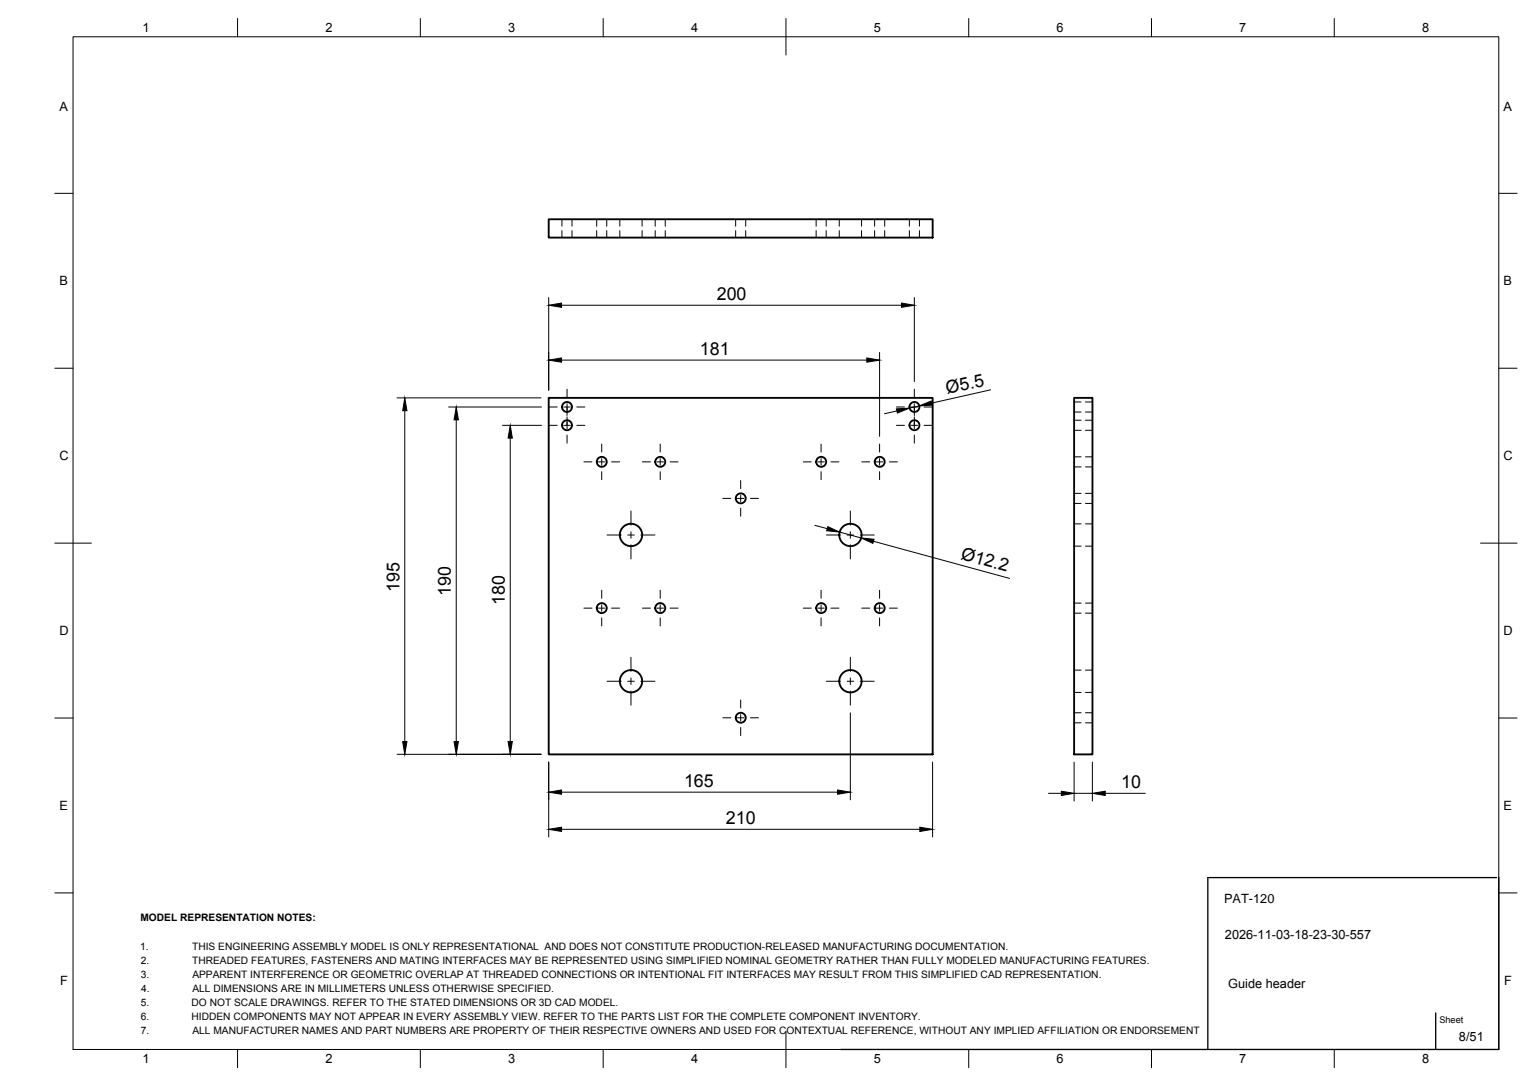
ISO-10303-21;
HEADER;
/* Generated by software containing ST-Developer
 * from STEP Tools, Inc. (www.steptools.com) 
 */

FILE_DESCRIPTION(
/* description */ ('Vibration shaker table dummy'),
/* implementation_level */ '2;1');

FILE_NAME(
/* name */ 'Guide header.step',
/* time_stamp */ '2026-10-27T10:55:14-07:00',
/* author */ (''),
/* organization */ (''),
/* preprocessor_version */ 'ST-DEVELOPER v20.2',
/* originating_system */ 'Autodesk Translation Framework v15.17.0.0',
/* authorisation */ '');

FILE_SCHEMA (('AUTOMOTIVE_DESIGN { 1 0 10303 214 3 1 1 }'));
ENDSEC;

DATA;
#10=MECHANICAL_DESIGN_GEOMETRIC_PRESENTATION_REPRESENTATION('',(#689),#22394);
#597=SHAPE_REPRESENTATION_RELATIONSHIP('SRR','None',#22643,#643);
#643=ADVANCED_BREP_SHAPE_REPRESENTATION('',(#735),#22349);
#689=STYLED_ITEM('',(#22947),#735);
#735=MANIFOLD_SOLID_BREP('Body1',#9207);
#819=FACE_BOUND('',#1946,.T.);
#820=FACE_BOUND('',#1947,.T.);
#821=FACE_BOUND('',#1948,.T.);
#822=FACE_BOUND('',#1949,.T.);
#823=FACE_BOUND('',#1950,.T.);
#824=FACE_BOUND('',#1951,.T.);
#825=FACE_BOUND('',#1952,.T.);
#826=FACE_BOUND('',#1953,.T.);
#827=FACE_BOUND('',#1954,.T.);
#828=FACE_BOUND('',#1955,.T.);
#829=FACE_BOUND('',#1956,.T.);
#830=FACE_BOUND('',#1957,.T.);
#831=FACE_BOUND('',#1958,.T.);
#832=FACE_BOUND('',#1959,.T.);
#833=FACE_BOUND('',#1960,.T.);
#834=FACE_BOUND('',#1961,.T.);
#835=FACE_BOUND('',#1962,.T.);
#836=FACE_BOUND('',#1963,.T.);
#837=FACE_BOUND('',#1965,.T.);
#838=FACE_BOUND('',#1966,.T.);
#839=FACE_BOUND('',#1967,.T.);
#840=FACE_BOUND('',#1968,.T.);
#841=FACE_BOUND('',#1969,.T.);
#842=FACE_BOUND('',#1970,.T.);
#843=FACE_BOUND('',#1971,.T.);
#844=FACE_BOUND('',#1972,.T.);
#845=FACE_BOUND('',#1973,.T.);
#846=FACE_BOUND('',#1974,.T.);
#847=FACE_BOUND('',#1975,.T.);
#848=FACE_BOUND('',#1976,.T.);
#849=FACE_BOUND('',#1977,.T.);
#850=FACE_BOUND('',#1978,.T.);
#851=FACE_BOUND('',#1979,.T.);
#852=FACE_BOUND('',#1980,.T.);
#853=FACE_BOUND('',#1981,.T.);
#854=FACE_BOUND('',#1982,.T.);
#1078=PLANE('',#9904);
#1079=PLANE('',#9905);
#1080=PLANE('',#9906);
#1081=PLANE('',#9907);
#1082=PLANE('',#9908);
#1083=PLANE('',#9909);
#1381=FACE_OUTER_BOUND('',#1923,.T.);
#1382=FACE_OUTER_BOUND('',#1924,.T.);
#1383=FACE_OUTER_BOUND('',#1925,.T.);
#1384=FACE_OUTER_BOUND('',#1926,.T.);
#1385=FACE_OUTER_BOUND('',#1927,.T.);
#1386=FACE_OUTER_BOUND('',#1928,.T.);
#1387=FACE_OUTER_BOUND('',#1929,.T.);
#1388=FACE_OUTER_BOUND('',#1930,.T.);
#1389=FACE_OUTER_BOUND('',#1931,.T.);
#1390=FACE_OUTER_BOUND('',#1932,.T.);
#1391=FACE_OUTER_BOUND('',#1933,.T.);
#1392=FACE_OUTER_BOUND('',#1934,.T.);
#1393=FACE_OUTER_BOUND('',#1935,.T.);
#1394=FACE_OUTER_BOUND('',#1936,.T.);
#1395=FACE_OUTER_BOUND('',#1937,.T.);
#1396=FACE_OUTER_BOUND('',#1938,.T.);
#1397=FACE_OUTER_BOUND('',#1939,.T.);
#1398=FACE_OUTER_BOUND('',#1940,.T.);
#1399=FACE_OUTER_BOUND('',#1941,.T.);
#1400=FACE_OUTER_BOUND('',#1942,.T.);
#1401=FACE_OUTER_BOUND('',#1943,.T.);
#1402=FACE_OUTER_BOUND('',#1944,.T.);
#1403=FACE_OUTER_BOUND('',#1945,.T.);
#1404=FACE_OUTER_BOUND('',#1964,.T.);
#1923=EDGE_LOOP('',(#6450,#6451,#6452,#6453));
#1924=EDGE_LOOP('',(#6454,#6455,#6456,#6457));
#1925=EDGE_LOOP('',(#6458,#6459,#6460,#6461));
#1926=EDGE_LOOP('',(#6462,#6463,#6464,#6465));
#1927=EDGE_LOOP('',(#6466,#6467,#6468,#6469));
#1928=EDGE_LOOP('',(#6470,#6471,#6472,#6473));
#1929=EDGE_LOOP('',(#6474,#6475,#6476,#6477));
#1930=EDGE_LOOP('',(#6478,#6479,#6480,#6481));
#1931=EDGE_LOOP('',(#6482,#6483,#6484,#6485));
#1932=EDGE_LOOP('',(#6486,#6487,#6488,#6489));
#1933=EDGE_LOOP('',(#6490,#6491,#6492,#6493));
#1934=EDGE_LOOP('',(#6494,#6495,#6496,#6497));
#1935=EDGE_LOOP('',(#6498,#6499,#6500,#6501));
#1936=EDGE_LOOP('',(#6502,#6503,#6504,#6505));
#1937=EDGE_LOOP('',(#6506,#6507,#6508,#6509));
#1938=EDGE_LOOP('',(#6510,#6511,#6512,#6513));
#1939=EDGE_LOOP('',(#6514,#6515,#6516,#6517));
#1940=EDGE_LOOP('',(#6518,#6519,#6520,#6521));
#1941=EDGE_LOOP('',(#6522,#6523,#6524,#6525));
#1942=EDGE_LOOP('',(#6526,#6527,#6528,#6529));
#1943=EDGE_LOOP('',(#6530,#6531,#6532,#6533));
#1944=EDGE_LOOP('',(#6534,#6535,#6536,#6537));
#1945=EDGE_LOOP('',(#6538,#6539,#6540,#6541));
#1946=EDGE_LOOP('',(#6542));
#1947=EDGE_LOOP('',(#6543));
#1948=EDGE_LOOP('',(#6544));
#1949=EDGE_LOOP('',(#6545));
#1950=EDGE_LOOP('',(#6546));
#1951=EDGE_LOOP('',(#6547));
#1952=EDGE_LOOP('',(#6548));
#1953=EDGE_LOOP('',(#6549));
#1954=EDGE_LOOP('',(#6550));
#1955=EDGE_LOOP('',(#6551));
#1956=EDGE_LOOP('',(#6552));
#1957=EDGE_LOOP('',(#6553));
#1958=EDGE_LOOP('',(#6554));
#1959=EDGE_LOOP('',(#6555));
#1960=EDGE_LOOP('',(#6556));
#1961=EDGE_LOOP('',(#6557));
#1962=EDGE_LOOP('',(#6558));
#1963=EDGE_LOOP('',(#6559));
#1964=EDGE_LOOP('',(#6560,#6561,#6562,#6563));
#1965=EDGE_LOOP('',(#6564));
#1966=EDGE_LOOP('',(#6565));
#1967=EDGE_LOOP('',(#6566));
#1968=EDGE_LOOP('',(#6567));
#1969=EDGE_LOOP('',(#6568));
#1970=EDGE_LOOP('',(#6569));
#1971=EDGE_LOOP('',(#6570));
#1972=EDGE_LOOP('',(#6571));
#1973=EDGE_LOOP('',(#6572));
#1974=EDGE_LOOP('',(#6573));
#1975=EDGE_LOOP('',(#6574));
#1976=EDGE_LOOP('',(#6575));
#1977=EDGE_LOOP('',(#6576));
#1978=EDGE_LOOP('',(#6577));
#1979=EDGE_LOOP('',(#6578));
#1980=EDGE_LOOP('',(#6579));
#1981=EDGE_LOOP('',(#6580));
#1982=EDGE_LOOP('',(#6581));
#2680=LINE('',#14169,#3299);
#2681=LINE('',#14175,#3300);
#2682=LINE('',#14181,#3301);
#2683=LINE('',#14187,#3302);
#2684=LINE('',#14193,#3303);
#2685=LINE('',#14199,#3304);
#2686=LINE('',#14205,#3305);
#2687=LINE('',#14211,#3306);
#2688=LINE('',#14217,#3307);
#2689=LINE('',#14223,#3308);
#2690=LINE('',#14229,#3309);
#2691=LINE('',#14235,#3310);
#2692=LINE('',#14241,#3311);
#2693=LINE('',#14247,#3312);
#2694=LINE('',#14253,#3313);
#2695=LINE('',#14259,#3314);
#2696=LINE('',#14265,#3315);
#2697=LINE('',#14271,#3316);
#2698=LINE('',#14276,#3317);
#2699=LINE('',#14278,#3318);
#2700=LINE('',#14280,#3319);
#2701=LINE('',#14281,#3320);
#2702=LINE('',#14284,#3321);
#2703=LINE('',#14286,#3322);
#2704=LINE('',#14287,#3323);
#2705=LINE('',#14290,#3324);
#2706=LINE('',#14292,#3325);
#2707=LINE('',#14293,#3326);
#2708=LINE('',#14295,#3327);
#2709=LINE('',#14296,#3328);
#3299=VECTOR('',#11192,0.275);
#3300=VECTOR('',#11199,0.275);
#3301=VECTOR('',#11206,0.275);
#3302=VECTOR('',#11213,0.275);
#3303=VECTOR('',#11220,0.275);
#3304=VECTOR('',#11227,0.275);
#3305=VECTOR('',#11234,0.275);
#3306=VECTOR('',#11241,0.275);
#3307=VECTOR('',#11248,0.275);
#3308=VECTOR('',#11255,0.275);
#3309=VECTOR('',#11262,0.275);
#3310=VECTOR('',#11269,0.275);
#3311=VECTOR('',#11276,0.275);
#3312=VECTOR('',#11283,0.275);
#3313=VECTOR('',#11290,0.61);
#3314=VECTOR('',#11297,0.61);
#3315=VECTOR('',#11304,0.61);
#3316=VECTOR('',#11311,0.61);
#3317=VECTOR('',#11316,1.);
#3318=VECTOR('',#11317,1.);
#3319=VECTOR('',#11318,1.);
#3320=VECTOR('',#11319,1.);
#3321=VECTOR('',#11322,1.);
#3322=VECTOR('',#11323,1.);
#3323=VECTOR('',#11324,1.);
#3324=VECTOR('',#11327,1.);
#3325=VECTOR('',#11328,1.);
#3326=VECTOR('',#11329,1.);
#3327=VECTOR('',#11332,1.);
#3328=VECTOR('',#11333,1.);
#3904=CIRCLE('',#9851,0.275);
#3905=CIRCLE('',#9852,0.275);
#3906=CIRCLE('',#9854,0.275);
#3907=CIRCLE('',#9855,0.275);
#3908=CIRCLE('',#9857,0.275);
#3909=CIRCLE('',#9858,0.275);
#3910=CIRCLE('',#9860,0.275);
#3911=CIRCLE('',#9861,0.275);
#3912=CIRCLE('',#9863,0.275);
#3913=CIRCLE('',#9864,0.275);
#3914=CIRCLE('',#9866,0.275);
#3915=CIRCLE('',#9867,0.275);
#3916=CIRCLE('',#9869,0.275);
#3917=CIRCLE('',#9870,0.275);
#3918=CIRCLE('',#9872,0.275);
#3919=CIRCLE('',#9873,0.275);
#3920=CIRCLE('',#9875,0.275);
#3921=CIRCLE('',#9876,0.275);
#3922=CIRCLE('',#9878,0.275);
#3923=CIRCLE('',#9879,0.275);
#3924=CIRCLE('',#9881,0.275);
#3925=CIRCLE('',#9882,0.275);
#3926=CIRCLE('',#9884,0.275);
#3927=CIRCLE('',#9885,0.275);
#3928=CIRCLE('',#9887,0.275);
#3929=CIRCLE('',#9888,0.275);
#3930=CIRCLE('',#9890,0.275);
#3931=CIRCLE('',#9891,0.275);
#3932=CIRCLE('',#9893,0.61);
#3933=CIRCLE('',#9894,0.61);
#3934=CIRCLE('',#9896,0.61);
#3935=CIRCLE('',#9897,0.61);
#3936=CIRCLE('',#9899,0.61);
#3937=CIRCLE('',#9900,0.61);
#3938=CIRCLE('',#9902,0.61);
#3939=CIRCLE('',#9903,0.61);
#4435=VERTEX_POINT('',#14166);
#4436=VERTEX_POINT('',#14168);
#4437=VERTEX_POINT('',#14172);
#4438=VERTEX_POINT('',#14174);
#4439=VERTEX_POINT('',#14178);
#4440=VERTEX_POINT('',#14180);
#4441=VERTEX_POINT('',#14184);
#4442=VERTEX_POINT('',#14186);
#4443=VERTEX_POINT('',#14190);
#4444=VERTEX_POINT('',#14192);
#4445=VERTEX_POINT('',#14196);
#4446=VERTEX_POINT('',#14198);
#4447=VERTEX_POINT('',#14202);
#4448=VERTEX_POINT('',#14204);
#4449=VERTEX_POINT('',#14208);
#4450=VERTEX_POINT('',#14210);
#4451=VERTEX_POINT('',#14214);
#4452=VERTEX_POINT('',#14216);
#4453=VERTEX_POINT('',#14220);
#4454=VERTEX_POINT('',#14222);
#4455=VERTEX_POINT('',#14226);
#4456=VERTEX_POINT('',#14228);
#4457=VERTEX_POINT('',#14232);
#4458=VERTEX_POINT('',#14234);
#4459=VERTEX_POINT('',#14238);
#4460=VERTEX_POINT('',#14240);
#4461=VERTEX_POINT('',#14244);
#4462=VERTEX_POINT('',#14246);
#4463=VERTEX_POINT('',#14250);
#4464=VERTEX_POINT('',#14252);
#4465=VERTEX_POINT('',#14256);
#4466=VERTEX_POINT('',#14258);
#4467=VERTEX_POINT('',#14262);
#4468=VERTEX_POINT('',#14264);
#4469=VERTEX_POINT('',#14268);
#4470=VERTEX_POINT('',#14270);
#4471=VERTEX_POINT('',#14274);
#4472=VERTEX_POINT('',#14275);
#4473=VERTEX_POINT('',#14277);
#4474=VERTEX_POINT('',#14279);
#4475=VERTEX_POINT('',#14283);
#4476=VERTEX_POINT('',#14285);
#4477=VERTEX_POINT('',#14289);
#4478=VERTEX_POINT('',#14291);
#5218=EDGE_CURVE('',#4435,#4435,#3904,.T.);
#5219=EDGE_CURVE('',#4435,#4436,#2680,.T.);
#5220=EDGE_CURVE('',#4436,#4436,#3905,.T.);
#5221=EDGE_CURVE('',#4437,#4437,#3906,.T.);
#5222=EDGE_CURVE('',#4437,#4438,#2681,.T.);
#5223=EDGE_CURVE('',#4438,#4438,#3907,.T.);
#5224=EDGE_CURVE('',#4439,#4439,#3908,.T.);
#5225=EDGE_CURVE('',#4439,#4440,#2682,.T.);
#5226=EDGE_CURVE('',#4440,#4440,#3909,.T.);
#5227=EDGE_CURVE('',#4441,#4441,#3910,.T.);
#5228=EDGE_CURVE('',#4441,#4442,#2683,.T.);
#5229=EDGE_CURVE('',#4442,#4442,#3911,.T.);
#5230=EDGE_CURVE('',#4443,#4443,#3912,.T.);
#5231=EDGE_CURVE('',#4443,#4444,#2684,.T.);
#5232=EDGE_CURVE('',#4444,#4444,#3913,.T.);
#5233=EDGE_CURVE('',#4445,#4445,#3914,.T.);
#5234=EDGE_CURVE('',#4445,#4446,#2685,.T.);
#5235=EDGE_CURVE('',#4446,#4446,#3915,.T.);
#5236=EDGE_CURVE('',#4447,#4447,#3916,.T.);
#5237=EDGE_CURVE('',#4447,#4448,#2686,.T.);
#5238=EDGE_CURVE('',#4448,#4448,#3917,.T.);
#5239=EDGE_CURVE('',#4449,#4449,#3918,.T.);
#5240=EDGE_CURVE('',#4449,#4450,#2687,.T.);
#5241=EDGE_CURVE('',#4450,#4450,#3919,.T.);
#5242=EDGE_CURVE('',#4451,#4451,#3920,.T.);
#5243=EDGE_CURVE('',#4451,#4452,#2688,.T.);
#5244=EDGE_CURVE('',#4452,#4452,#3921,.T.);
#5245=EDGE_CURVE('',#4453,#4453,#3922,.T.);
#5246=EDGE_CURVE('',#4453,#4454,#2689,.T.);
#5247=EDGE_CURVE('',#4454,#4454,#3923,.T.);
#5248=EDGE_CURVE('',#4455,#4455,#3924,.T.);
#5249=EDGE_CURVE('',#4455,#4456,#2690,.T.);
#5250=EDGE_CURVE('',#4456,#4456,#3925,.T.);
#5251=EDGE_CURVE('',#4457,#4457,#3926,.T.);
#5252=EDGE_CURVE('',#4457,#4458,#2691,.T.);
#5253=EDGE_CURVE('',#4458,#4458,#3927,.T.);
#5254=EDGE_CURVE('',#4459,#4459,#3928,.T.);
#5255=EDGE_CURVE('',#4459,#4460,#2692,.T.);
#5256=EDGE_CURVE('',#4460,#4460,#3929,.T.);
#5257=EDGE_CURVE('',#4461,#4461,#3930,.T.);
#5258=EDGE_CURVE('',#4461,#4462,#2693,.T.);
#5259=EDGE_CURVE('',#4462,#4462,#3931,.T.);
#5260=EDGE_CURVE('',#4463,#4463,#3932,.T.);
#5261=EDGE_CURVE('',#4463,#4464,#2694,.T.);
#5262=EDGE_CURVE('',#4464,#4464,#3933,.T.);
#5263=EDGE_CURVE('',#4465,#4465,#3934,.T.);
#5264=EDGE_CURVE('',#4465,#4466,#2695,.T.);
#5265=EDGE_CURVE('',#4466,#4466,#3935,.T.);
#5266=EDGE_CURVE('',#4467,#4467,#3936,.T.);
#5267=EDGE_CURVE('',#4467,#4468,#2696,.T.);
#5268=EDGE_CURVE('',#4468,#4468,#3937,.T.);
#5269=EDGE_CURVE('',#4469,#4469,#3938,.T.);
#5270=EDGE_CURVE('',#4469,#4470,#2697,.T.);
#5271=EDGE_CURVE('',#4470,#4470,#3939,.T.);
#5272=EDGE_CURVE('',#4471,#4472,#2698,.T.);
#5273=EDGE_CURVE('',#4472,#4473,#2699,.T.);
#5274=EDGE_CURVE('',#4474,#4473,#2700,.T.);
#5275=EDGE_CURVE('',#4471,#4474,#2701,.T.);
#5276=EDGE_CURVE('',#4475,#4471,#2702,.T.);
#5277=EDGE_CURVE('',#4476,#4474,#2703,.T.);
#5278=EDGE_CURVE('',#4475,#4476,#2704,.T.);
#5279=EDGE_CURVE('',#4477,#4475,#2705,.T.);
#5280=EDGE_CURVE('',#4478,#4476,#2706,.T.);
#5281=EDGE_CURVE('',#4477,#4478,#2707,.T.);
#5282=EDGE_CURVE('',#4472,#4477,#2708,.T.);
#5283=EDGE_CURVE('',#4473,#4478,#2709,.T.);
#6450=ORIENTED_EDGE('',*,*,#5218,.F.);
#6451=ORIENTED_EDGE('',*,*,#5219,.T.);
#6452=ORIENTED_EDGE('',*,*,#5220,.F.);
#6453=ORIENTED_EDGE('',*,*,#5219,.F.);
#6454=ORIENTED_EDGE('',*,*,#5221,.F.);
#6455=ORIENTED_EDGE('',*,*,#5222,.T.);
#6456=ORIENTED_EDGE('',*,*,#5223,.F.);
#6457=ORIENTED_EDGE('',*,*,#5222,.F.);
#6458=ORIENTED_EDGE('',*,*,#5224,.F.);
#6459=ORIENTED_EDGE('',*,*,#5225,.T.);
#6460=ORIENTED_EDGE('',*,*,#5226,.F.);
#6461=ORIENTED_EDGE('',*,*,#5225,.F.);
#6462=ORIENTED_EDGE('',*,*,#5227,.F.);
#6463=ORIENTED_EDGE('',*,*,#5228,.T.);
#6464=ORIENTED_EDGE('',*,*,#5229,.F.);
#6465=ORIENTED_EDGE('',*,*,#5228,.F.);
#6466=ORIENTED_EDGE('',*,*,#5230,.F.);
#6467=ORIENTED_EDGE('',*,*,#5231,.T.);
#6468=ORIENTED_EDGE('',*,*,#5232,.F.);
#6469=ORIENTED_EDGE('',*,*,#5231,.F.);
#6470=ORIENTED_EDGE('',*,*,#5233,.F.);
#6471=ORIENTED_EDGE('',*,*,#5234,.T.);
#6472=ORIENTED_EDGE('',*,*,#5235,.F.);
#6473=ORIENTED_EDGE('',*,*,#5234,.F.);
#6474=ORIENTED_EDGE('',*,*,#5236,.F.);
#6475=ORIENTED_EDGE('',*,*,#5237,.T.);
#6476=ORIENTED_EDGE('',*,*,#5238,.F.);
#6477=ORIENTED_EDGE('',*,*,#5237,.F.);
#6478=ORIENTED_EDGE('',*,*,#5239,.F.);
#6479=ORIENTED_EDGE('',*,*,#5240,.T.);
#6480=ORIENTED_EDGE('',*,*,#5241,.F.);
#6481=ORIENTED_EDGE('',*,*,#5240,.F.);
#6482=ORIENTED_EDGE('',*,*,#5242,.F.);
#6483=ORIENTED_EDGE('',*,*,#5243,.T.);
#6484=ORIENTED_EDGE('',*,*,#5244,.F.);
#6485=ORIENTED_EDGE('',*,*,#5243,.F.);
#6486=ORIENTED_EDGE('',*,*,#5245,.F.);
#6487=ORIENTED_EDGE('',*,*,#5246,.T.);
#6488=ORIENTED_EDGE('',*,*,#5247,.F.);
#6489=ORIENTED_EDGE('',*,*,#5246,.F.);
#6490=ORIENTED_EDGE('',*,*,#5248,.F.);
#6491=ORIENTED_EDGE('',*,*,#5249,.T.);
#6492=ORIENTED_EDGE('',*,*,#5250,.F.);
#6493=ORIENTED_EDGE('',*,*,#5249,.F.);
#6494=ORIENTED_EDGE('',*,*,#5251,.F.);
#6495=ORIENTED_EDGE('',*,*,#5252,.T.);
#6496=ORIENTED_EDGE('',*,*,#5253,.F.);
#6497=ORIENTED_EDGE('',*,*,#5252,.F.);
#6498=ORIENTED_EDGE('',*,*,#5254,.F.);
#6499=ORIENTED_EDGE('',*,*,#5255,.T.);
#6500=ORIENTED_EDGE('',*,*,#5256,.F.);
#6501=ORIENTED_EDGE('',*,*,#5255,.F.);
#6502=ORIENTED_EDGE('',*,*,#5257,.F.);
#6503=ORIENTED_EDGE('',*,*,#5258,.T.);
#6504=ORIENTED_EDGE('',*,*,#5259,.F.);
#6505=ORIENTED_EDGE('',*,*,#5258,.F.);
#6506=ORIENTED_EDGE('',*,*,#5260,.F.);
#6507=ORIENTED_EDGE('',*,*,#5261,.T.);
#6508=ORIENTED_EDGE('',*,*,#5262,.F.);
#6509=ORIENTED_EDGE('',*,*,#5261,.F.);
#6510=ORIENTED_EDGE('',*,*,#5263,.F.);
#6511=ORIENTED_EDGE('',*,*,#5264,.T.);
#6512=ORIENTED_EDGE('',*,*,#5265,.F.);
#6513=ORIENTED_EDGE('',*,*,#5264,.F.);
#6514=ORIENTED_EDGE('',*,*,#5266,.F.);
#6515=ORIENTED_EDGE('',*,*,#5267,.T.);
#6516=ORIENTED_EDGE('',*,*,#5268,.F.);
#6517=ORIENTED_EDGE('',*,*,#5267,.F.);
#6518=ORIENTED_EDGE('',*,*,#5269,.F.);
#6519=ORIENTED_EDGE('',*,*,#5270,.T.);
#6520=ORIENTED_EDGE('',*,*,#5271,.F.);
#6521=ORIENTED_EDGE('',*,*,#5270,.F.);
#6522=ORIENTED_EDGE('',*,*,#5272,.T.);
#6523=ORIENTED_EDGE('',*,*,#5273,.T.);
#6524=ORIENTED_EDGE('',*,*,#5274,.F.);
#6525=ORIENTED_EDGE('',*,*,#5275,.F.);
#6526=ORIENTED_EDGE('',*,*,#5276,.T.);
#6527=ORIENTED_EDGE('',*,*,#5275,.T.);
#6528=ORIENTED_EDGE('',*,*,#5277,.F.);
#6529=ORIENTED_EDGE('',*,*,#5278,.F.);
#6530=ORIENTED_EDGE('',*,*,#5279,.T.);
#6531=ORIENTED_EDGE('',*,*,#5278,.T.);
#6532=ORIENTED_EDGE('',*,*,#5280,.F.);
#6533=ORIENTED_EDGE('',*,*,#5281,.F.);
#6534=ORIENTED_EDGE('',*,*,#5282,.T.);
#6535=ORIENTED_EDGE('',*,*,#5281,.T.);
#6536=ORIENTED_EDGE('',*,*,#5283,.F.);
#6537=ORIENTED_EDGE('',*,*,#5273,.F.);
#6538=ORIENTED_EDGE('',*,*,#5283,.T.);
#6539=ORIENTED_EDGE('',*,*,#5280,.T.);
#6540=ORIENTED_EDGE('',*,*,#5277,.T.);
#6541=ORIENTED_EDGE('',*,*,#5274,.T.);
#6542=ORIENTED_EDGE('',*,*,#5223,.T.);
#6543=ORIENTED_EDGE('',*,*,#5232,.T.);
#6544=ORIENTED_EDGE('',*,*,#5235,.T.);
#6545=ORIENTED_EDGE('',*,*,#5244,.T.);
#6546=ORIENTED_EDGE('',*,*,#5247,.T.);
#6547=ORIENTED_EDGE('',*,*,#5271,.T.);
#6548=ORIENTED_EDGE('',*,*,#5268,.T.);
#6549=ORIENTED_EDGE('',*,*,#5265,.T.);
#6550=ORIENTED_EDGE('',*,*,#5262,.T.);
#6551=ORIENTED_EDGE('',*,*,#5259,.T.);
#6552=ORIENTED_EDGE('',*,*,#5256,.T.);
#6553=ORIENTED_EDGE('',*,*,#5253,.T.);
#6554=ORIENTED_EDGE('',*,*,#5250,.T.);
#6555=ORIENTED_EDGE('',*,*,#5241,.T.);
#6556=ORIENTED_EDGE('',*,*,#5238,.T.);
#6557=ORIENTED_EDGE('',*,*,#5229,.T.);
#6558=ORIENTED_EDGE('',*,*,#5226,.T.);
#6559=ORIENTED_EDGE('',*,*,#5220,.T.);
#6560=ORIENTED_EDGE('',*,*,#5282,.F.);
#6561=ORIENTED_EDGE('',*,*,#5272,.F.);
#6562=ORIENTED_EDGE('',*,*,#5276,.F.);
#6563=ORIENTED_EDGE('',*,*,#5279,.F.);
#6564=ORIENTED_EDGE('',*,*,#5221,.T.);
#6565=ORIENTED_EDGE('',*,*,#5230,.T.);
#6566=ORIENTED_EDGE('',*,*,#5233,.T.);
#6567=ORIENTED_EDGE('',*,*,#5242,.T.);
#6568=ORIENTED_EDGE('',*,*,#5245,.T.);
#6569=ORIENTED_EDGE('',*,*,#5269,.T.);
#6570=ORIENTED_EDGE('',*,*,#5266,.T.);
#6571=ORIENTED_EDGE('',*,*,#5263,.T.);
#6572=ORIENTED_EDGE('',*,*,#5260,.T.);
#6573=ORIENTED_EDGE('',*,*,#5257,.T.);
#6574=ORIENTED_EDGE('',*,*,#5254,.T.);
#6575=ORIENTED_EDGE('',*,*,#5251,.T.);
#6576=ORIENTED_EDGE('',*,*,#5248,.T.);
#6577=ORIENTED_EDGE('',*,*,#5239,.T.);
#6578=ORIENTED_EDGE('',*,*,#5236,.T.);
#6579=ORIENTED_EDGE('',*,*,#5227,.T.);
#6580=ORIENTED_EDGE('',*,*,#5224,.T.);
#6581=ORIENTED_EDGE('',*,*,#5218,.T.);
#8528=CYLINDRICAL_SURFACE('',#9850,0.275);
#8529=CYLINDRICAL_SURFACE('',#9853,0.275);
#8530=CYLINDRICAL_SURFACE('',#9856,0.275);
#8531=CYLINDRICAL_SURFACE('',#9859,0.275);
#8532=CYLINDRICAL_SURFACE('',#9862,0.275);
#8533=CYLINDRICAL_SURFACE('',#9865,0.275);
#8534=CYLINDRICAL_SURFACE('',#9868,0.275);
#8535=CYLINDRICAL_SURFACE('',#9871,0.275);
#8536=CYLINDRICAL_SURFACE('',#9874,0.275);
#8537=CYLINDRICAL_SURFACE('',#9877,0.275);
#8538=CYLINDRICAL_SURFACE('',#9880,0.275);
#8539=CYLINDRICAL_SURFACE('',#9883,0.275);
#8540=CYLINDRICAL_SURFACE('',#9886,0.275);
#8541=CYLINDRICAL_SURFACE('',#9889,0.275);
#8542=CYLINDRICAL_SURFACE('',#9892,0.61);
#8543=CYLINDRICAL_SURFACE('',#9895,0.61);
#8544=CYLINDRICAL_SURFACE('',#9898,0.61);
#8545=CYLINDRICAL_SURFACE('',#9901,0.61);
#8746=ADVANCED_FACE('',(#1381),#8528,.F.);
#8747=ADVANCED_FACE('',(#1382),#8529,.F.);
#8748=ADVANCED_FACE('',(#1383),#8530,.F.);
#8749=ADVANCED_FACE('',(#1384),#8531,.F.);
#8750=ADVANCED_FACE('',(#1385),#8532,.F.);
#8751=ADVANCED_FACE('',(#1386),#8533,.F.);
#8752=ADVANCED_FACE('',(#1387),#8534,.F.);
#8753=ADVANCED_FACE('',(#1388),#8535,.F.);
#8754=ADVANCED_FACE('',(#1389),#8536,.F.);
#8755=ADVANCED_FACE('',(#1390),#8537,.F.);
#8756=ADVANCED_FACE('',(#1391),#8538,.F.);
#8757=ADVANCED_FACE('',(#1392),#8539,.F.);
#8758=ADVANCED_FACE('',(#1393),#8540,.F.);
#8759=ADVANCED_FACE('',(#1394),#8541,.F.);
#8760=ADVANCED_FACE('',(#1395),#8542,.F.);
#8761=ADVANCED_FACE('',(#1396),#8543,.F.);
#8762=ADVANCED_FACE('',(#1397),#8544,.F.);
#8763=ADVANCED_FACE('',(#1398),#8545,.F.);
#8764=ADVANCED_FACE('',(#1399),#1078,.T.);
#8765=ADVANCED_FACE('',(#1400),#1079,.T.);
#8766=ADVANCED_FACE('',(#1401),#1080,.T.);
#8767=ADVANCED_FACE('',(#1402),#1081,.T.);
#8768=ADVANCED_FACE('',(#1403,#819,#820,#821,#822,#823,#824,#825,#826,#827,
#828,#829,#830,#831,#832,#833,#834,#835,#836),#1082,.T.);
#8769=ADVANCED_FACE('',(#1404,#837,#838,#839,#840,#841,#842,#843,#844,#845,
#846,#847,#848,#849,#850,#851,#852,#853,#854),#1083,.F.);
#9207=CLOSED_SHELL('',(#8746,#8747,#8748,#8749,#8750,#8751,#8752,#8753,
#8754,#8755,#8756,#8757,#8758,#8759,#8760,#8761,#8762,#8763,#8764,#8765,
#8766,#8767,#8768,#8769));
#9849=AXIS2_PLACEMENT_3D('',#14164,#11186,#11187);
#9850=AXIS2_PLACEMENT_3D('',#14165,#11188,#11189);
#9851=AXIS2_PLACEMENT_3D('',#14167,#11190,#11191);
#9852=AXIS2_PLACEMENT_3D('',#14170,#11193,#11194);
#9853=AXIS2_PLACEMENT_3D('',#14171,#11195,#11196);
#9854=AXIS2_PLACEMENT_3D('',#14173,#11197,#11198);
#9855=AXIS2_PLACEMENT_3D('',#14176,#11200,#11201);
#9856=AXIS2_PLACEMENT_3D('',#14177,#11202,#11203);
#9857=AXIS2_PLACEMENT_3D('',#14179,#11204,#11205);
#9858=AXIS2_PLACEMENT_3D('',#14182,#11207,#11208);
#9859=AXIS2_PLACEMENT_3D('',#14183,#11209,#11210);
#9860=AXIS2_PLACEMENT_3D('',#14185,#11211,#11212);
#9861=AXIS2_PLACEMENT_3D('',#14188,#11214,#11215);
#9862=AXIS2_PLACEMENT_3D('',#14189,#11216,#11217);
#9863=AXIS2_PLACEMENT_3D('',#14191,#11218,#11219);
#9864=AXIS2_PLACEMENT_3D('',#14194,#11221,#11222);
#9865=AXIS2_PLACEMENT_3D('',#14195,#11223,#11224);
#9866=AXIS2_PLACEMENT_3D('',#14197,#11225,#11226);
#9867=AXIS2_PLACEMENT_3D('',#14200,#11228,#11229);
#9868=AXIS2_PLACEMENT_3D('',#14201,#11230,#11231);
#9869=AXIS2_PLACEMENT_3D('',#14203,#11232,#11233);
#9870=AXIS2_PLACEMENT_3D('',#14206,#11235,#11236);
#9871=AXIS2_PLACEMENT_3D('',#14207,#11237,#11238);
#9872=AXIS2_PLACEMENT_3D('',#14209,#11239,#11240);
#9873=AXIS2_PLACEMENT_3D('',#14212,#11242,#11243);
#9874=AXIS2_PLACEMENT_3D('',#14213,#11244,#11245);
#9875=AXIS2_PLACEMENT_3D('',#14215,#11246,#11247);
#9876=AXIS2_PLACEMENT_3D('',#14218,#11249,#11250);
#9877=AXIS2_PLACEMENT_3D('',#14219,#11251,#11252);
#9878=AXIS2_PLACEMENT_3D('',#14221,#11253,#11254);
#9879=AXIS2_PLACEMENT_3D('',#14224,#11256,#11257);
#9880=AXIS2_PLACEMENT_3D('',#14225,#11258,#11259);
#9881=AXIS2_PLACEMENT_3D('',#14227,#11260,#11261);
#9882=AXIS2_PLACEMENT_3D('',#14230,#11263,#11264);
#9883=AXIS2_PLACEMENT_3D('',#14231,#11265,#11266);
#9884=AXIS2_PLACEMENT_3D('',#14233,#11267,#11268);
#9885=AXIS2_PLACEMENT_3D('',#14236,#11270,#11271);
#9886=AXIS2_PLACEMENT_3D('',#14237,#11272,#11273);
#9887=AXIS2_PLACEMENT_3D('',#14239,#11274,#11275);
#9888=AXIS2_PLACEMENT_3D('',#14242,#11277,#11278);
#9889=AXIS2_PLACEMENT_3D('',#14243,#11279,#11280);
#9890=AXIS2_PLACEMENT_3D('',#14245,#11281,#11282);
#9891=AXIS2_PLACEMENT_3D('',#14248,#11284,#11285);
#9892=AXIS2_PLACEMENT_3D('',#14249,#11286,#11287);
#9893=AXIS2_PLACEMENT_3D('',#14251,#11288,#11289);
#9894=AXIS2_PLACEMENT_3D('',#14254,#11291,#11292);
#9895=AXIS2_PLACEMENT_3D('',#14255,#11293,#11294);
#9896=AXIS2_PLACEMENT_3D('',#14257,#11295,#11296);
#9897=AXIS2_PLACEMENT_3D('',#14260,#11298,#11299);
#9898=AXIS2_PLACEMENT_3D('',#14261,#11300,#11301);
#9899=AXIS2_PLACEMENT_3D('',#14263,#11302,#11303);
#9900=AXIS2_PLACEMENT_3D('',#14266,#11305,#11306);
#9901=AXIS2_PLACEMENT_3D('',#14267,#11307,#11308);
#9902=AXIS2_PLACEMENT_3D('',#14269,#11309,#11310);
#9903=AXIS2_PLACEMENT_3D('',#14272,#11312,#11313);
#9904=AXIS2_PLACEMENT_3D('',#14273,#11314,#11315);
#9905=AXIS2_PLACEMENT_3D('',#14282,#11320,#11321);
#9906=AXIS2_PLACEMENT_3D('',#14288,#11325,#11326);
#9907=AXIS2_PLACEMENT_3D('',#14294,#11330,#11331);
#9908=AXIS2_PLACEMENT_3D('',#14297,#11334,#11335);
#9909=AXIS2_PLACEMENT_3D('',#14298,#11336,#11337);
#11186=DIRECTION('axis',(0.,0.,1.));
#11187=DIRECTION('refdir',(1.,0.,0.));
#11188=DIRECTION('center_axis',(0.,0.,1.));
#11189=DIRECTION('ref_axis',(1.,0.,0.));
#11190=DIRECTION('center_axis',(0.,0.,1.));
#11191=DIRECTION('ref_axis',(1.,0.,0.));
#11192=DIRECTION('',(0.,0.,1.));
#11193=DIRECTION('center_axis',(0.,0.,-1.));
#11194=DIRECTION('ref_axis',(1.,0.,0.));
#11195=DIRECTION('center_axis',(0.,0.,1.));
#11196=DIRECTION('ref_axis',(1.,0.,0.));
#11197=DIRECTION('center_axis',(0.,0.,1.));
#11198=DIRECTION('ref_axis',(1.,0.,0.));
#11199=DIRECTION('',(0.,0.,1.));
#11200=DIRECTION('center_axis',(0.,0.,-1.));
#11201=DIRECTION('ref_axis',(1.,0.,0.));
#11202=DIRECTION('center_axis',(0.,0.,1.));
#11203=DIRECTION('ref_axis',(1.,0.,0.));
#11204=DIRECTION('center_axis',(0.,0.,1.));
#11205=DIRECTION('ref_axis',(1.,0.,0.));
#11206=DIRECTION('',(0.,0.,1.));
#11207=DIRECTION('center_axis',(0.,0.,-1.));
#11208=DIRECTION('ref_axis',(1.,0.,0.));
#11209=DIRECTION('center_axis',(0.,0.,1.));
#11210=DIRECTION('ref_axis',(1.,0.,0.));
#11211=DIRECTION('center_axis',(0.,0.,1.));
#11212=DIRECTION('ref_axis',(1.,0.,0.));
#11213=DIRECTION('',(0.,0.,1.));
#11214=DIRECTION('center_axis',(0.,0.,-1.));
#11215=DIRECTION('ref_axis',(1.,0.,0.));
#11216=DIRECTION('center_axis',(0.,0.,1.));
#11217=DIRECTION('ref_axis',(1.,0.,0.));
#11218=DIRECTION('center_axis',(0.,0.,1.));
#11219=DIRECTION('ref_axis',(1.,0.,0.));
#11220=DIRECTION('',(0.,0.,1.));
#11221=DIRECTION('center_axis',(0.,0.,-1.));
#11222=DIRECTION('ref_axis',(1.,0.,0.));
#11223=DIRECTION('center_axis',(0.,0.,1.));
#11224=DIRECTION('ref_axis',(1.,0.,0.));
#11225=DIRECTION('center_axis',(0.,0.,1.));
#11226=DIRECTION('ref_axis',(1.,0.,0.));
#11227=DIRECTION('',(0.,0.,1.));
#11228=DIRECTION('center_axis',(0.,0.,-1.));
#11229=DIRECTION('ref_axis',(1.,0.,0.));
#11230=DIRECTION('center_axis',(0.,0.,1.));
#11231=DIRECTION('ref_axis',(1.,0.,0.));
#11232=DIRECTION('center_axis',(0.,0.,1.));
#11233=DIRECTION('ref_axis',(1.,0.,0.));
#11234=DIRECTION('',(0.,0.,1.));
#11235=DIRECTION('center_axis',(0.,0.,-1.));
#11236=DIRECTION('ref_axis',(1.,0.,0.));
#11237=DIRECTION('center_axis',(0.,0.,1.));
#11238=DIRECTION('ref_axis',(1.,0.,0.));
#11239=DIRECTION('center_axis',(0.,0.,1.));
#11240=DIRECTION('ref_axis',(1.,0.,0.));
#11241=DIRECTION('',(0.,0.,1.));
#11242=DIRECTION('center_axis',(0.,0.,-1.));
#11243=DIRECTION('ref_axis',(1.,0.,0.));
#11244=DIRECTION('center_axis',(0.,0.,1.));
#11245=DIRECTION('ref_axis',(1.,0.,0.));
#11246=DIRECTION('center_axis',(0.,0.,1.));
#11247=DIRECTION('ref_axis',(1.,0.,0.));
#11248=DIRECTION('',(0.,0.,1.));
#11249=DIRECTION('center_axis',(0.,0.,-1.));
#11250=DIRECTION('ref_axis',(1.,0.,0.));
#11251=DIRECTION('center_axis',(0.,0.,1.));
#11252=DIRECTION('ref_axis',(1.,0.,0.));
#11253=DIRECTION('center_axis',(0.,0.,1.));
#11254=DIRECTION('ref_axis',(1.,0.,0.));
#11255=DIRECTION('',(0.,0.,1.));
#11256=DIRECTION('center_axis',(0.,0.,-1.));
#11257=DIRECTION('ref_axis',(1.,0.,0.));
#11258=DIRECTION('center_axis',(0.,0.,1.));
#11259=DIRECTION('ref_axis',(1.,0.,0.));
#11260=DIRECTION('center_axis',(0.,0.,1.));
#11261=DIRECTION('ref_axis',(1.,0.,0.));
#11262=DIRECTION('',(0.,0.,1.));
#11263=DIRECTION('center_axis',(0.,0.,-1.));
#11264=DIRECTION('ref_axis',(1.,0.,0.));
#11265=DIRECTION('center_axis',(0.,0.,1.));
#11266=DIRECTION('ref_axis',(1.,0.,0.));
#11267=DIRECTION('center_axis',(0.,0.,1.));
#11268=DIRECTION('ref_axis',(1.,0.,0.));
#11269=DIRECTION('',(0.,0.,1.));
#11270=DIRECTION('center_axis',(0.,0.,-1.));
#11271=DIRECTION('ref_axis',(1.,0.,0.));
#11272=DIRECTION('center_axis',(0.,0.,1.));
#11273=DIRECTION('ref_axis',(1.,0.,0.));
#11274=DIRECTION('center_axis',(0.,0.,1.));
#11275=DIRECTION('ref_axis',(1.,0.,0.));
#11276=DIRECTION('',(0.,0.,1.));
#11277=DIRECTION('center_axis',(0.,0.,-1.));
#11278=DIRECTION('ref_axis',(1.,0.,0.));
#11279=DIRECTION('center_axis',(0.,0.,1.));
#11280=DIRECTION('ref_axis',(1.,0.,0.));
#11281=DIRECTION('center_axis',(0.,0.,1.));
#11282=DIRECTION('ref_axis',(1.,0.,0.));
#11283=DIRECTION('',(0.,0.,1.));
#11284=DIRECTION('center_axis',(0.,0.,-1.));
#11285=DIRECTION('ref_axis',(1.,0.,0.));
#11286=DIRECTION('center_axis',(0.,0.,1.));
#11287=DIRECTION('ref_axis',(1.,0.,0.));
#11288=DIRECTION('center_axis',(0.,0.,1.));
#11289=DIRECTION('ref_axis',(1.,0.,0.));
#11290=DIRECTION('',(0.,0.,1.));
#11291=DIRECTION('center_axis',(0.,0.,-1.));
#11292=DIRECTION('ref_axis',(1.,0.,0.));
#11293=DIRECTION('center_axis',(0.,0.,1.));
#11294=DIRECTION('ref_axis',(1.,0.,0.));
#11295=DIRECTION('center_axis',(0.,0.,1.));
#11296=DIRECTION('ref_axis',(1.,0.,0.));
#11297=DIRECTION('',(0.,0.,1.));
#11298=DIRECTION('center_axis',(0.,0.,-1.));
#11299=DIRECTION('ref_axis',(1.,0.,0.));
#11300=DIRECTION('center_axis',(0.,0.,1.));
#11301=DIRECTION('ref_axis',(1.,0.,0.));
#11302=DIRECTION('center_axis',(0.,0.,1.));
#11303=DIRECTION('ref_axis',(1.,0.,0.));
#11304=DIRECTION('',(0.,0.,1.));
#11305=DIRECTION('center_axis',(0.,0.,-1.));
#11306=DIRECTION('ref_axis',(1.,0.,0.));
#11307=DIRECTION('center_axis',(0.,0.,1.));
#11308=DIRECTION('ref_axis',(1.,0.,0.));
#11309=DIRECTION('center_axis',(0.,0.,1.));
#11310=DIRECTION('ref_axis',(1.,0.,0.));
#11311=DIRECTION('',(0.,0.,1.));
#11312=DIRECTION('center_axis',(0.,0.,-1.));
#11313=DIRECTION('ref_axis',(1.,0.,0.));
#11314=DIRECTION('center_axis',(0.,1.,0.));
#11315=DIRECTION('ref_axis',(-1.,0.,0.));
#11316=DIRECTION('',(-1.,0.,0.));
#11317=DIRECTION('',(0.,0.,1.));
#11318=DIRECTION('',(-1.,0.,0.));
#11319=DIRECTION('',(0.,0.,1.));
#11320=DIRECTION('center_axis',(1.,0.,0.));
#11321=DIRECTION('ref_axis',(0.,1.,0.));
#11322=DIRECTION('',(0.,1.,0.));
#11323=DIRECTION('',(0.,1.,0.));
#11324=DIRECTION('',(0.,0.,1.));
#11325=DIRECTION('center_axis',(0.,-1.,0.));
#11326=DIRECTION('ref_axis',(1.,0.,0.));
#11327=DIRECTION('',(1.,0.,0.));
#11328=DIRECTION('',(1.,0.,0.));
#11329=DIRECTION('',(0.,0.,1.));
#11330=DIRECTION('center_axis',(-1.,0.,0.));
#11331=DIRECTION('ref_axis',(0.,-1.,0.));
#11332=DIRECTION('',(0.,-1.,0.));
#11333=DIRECTION('',(0.,-1.,0.));
#11334=DIRECTION('center_axis',(0.,0.,1.));
#11335=DIRECTION('ref_axis',(1.,0.,0.));
#11336=DIRECTION('center_axis',(0.,0.,1.));
#11337=DIRECTION('ref_axis',(1.,0.,0.));
#14164=CARTESIAN_POINT('',(0.,0.,0.));
#14165=CARTESIAN_POINT('Origin',(0.,6.,30.4));
#14166=CARTESIAN_POINT('',(-0.275,6.,30.5));
#14167=CARTESIAN_POINT('Origin',(0.,6.,30.5));
#14168=CARTESIAN_POINT('',(-0.275,6.,31.5));
#14169=CARTESIAN_POINT('',(-0.275,6.,30.4));
#14170=CARTESIAN_POINT('Origin',(0.,6.,31.5));
#14171=CARTESIAN_POINT('Origin',(0.,-6.,30.4));
#14172=CARTESIAN_POINT('',(-0.275,-6.,30.5));
#14173=CARTESIAN_POINT('Origin',(0.,-6.,30.5));
#14174=CARTESIAN_POINT('',(-0.275,-6.,31.5));
#14175=CARTESIAN_POINT('',(-0.275,-6.,30.4));
#14176=CARTESIAN_POINT('Origin',(0.,-6.,31.5));
#14177=CARTESIAN_POINT('Origin',(4.4,8.,30.4));
#14178=CARTESIAN_POINT('',(4.125,8.,30.5));
#14179=CARTESIAN_POINT('Origin',(4.4,8.,30.5));
#14180=CARTESIAN_POINT('',(4.125,8.,31.5));
#14181=CARTESIAN_POINT('',(4.125,8.,30.4));
#14182=CARTESIAN_POINT('Origin',(4.4,8.,31.5));
#14183=CARTESIAN_POINT('Origin',(7.6,8.,30.4));
#14184=CARTESIAN_POINT('',(7.325,8.,30.5));
#14185=CARTESIAN_POINT('Origin',(7.6,8.,30.5));
#14186=CARTESIAN_POINT('',(7.325,8.,31.5));
#14187=CARTESIAN_POINT('',(7.325,8.,30.4));
#14188=CARTESIAN_POINT('Origin',(7.6,8.,31.5));
#14189=CARTESIAN_POINT('Origin',(4.4,0.,30.4));
#14190=CARTESIAN_POINT('',(4.125,-3.36777869765523E-17,30.5));
#14191=CARTESIAN_POINT('Origin',(4.4,0.,30.5));
#14192=CARTESIAN_POINT('',(4.125,3.36777869765523E-17,31.5));
#14193=CARTESIAN_POINT('',(4.125,-3.36777869765523E-17,30.4));
#14194=CARTESIAN_POINT('Origin',(4.4,0.,31.5));
#14195=CARTESIAN_POINT('Origin',(7.6,0.,30.4));
#14196=CARTESIAN_POINT('',(7.325,-3.36777869765523E-17,30.5));
#14197=CARTESIAN_POINT('Origin',(7.6,0.,30.5));
#14198=CARTESIAN_POINT('',(7.325,3.36777869765523E-17,31.5));
#14199=CARTESIAN_POINT('',(7.325,-3.36777869765523E-17,30.4));
#14200=CARTESIAN_POINT('Origin',(7.6,0.,31.5));
#14201=CARTESIAN_POINT('Origin',(-7.6,8.,30.4));
#14202=CARTESIAN_POINT('',(-7.875,8.,30.5));
#14203=CARTESIAN_POINT('Origin',(-7.6,8.,30.5));
#14204=CARTESIAN_POINT('',(-7.875,8.,31.5));
#14205=CARTESIAN_POINT('',(-7.875,8.,30.4));
#14206=CARTESIAN_POINT('Origin',(-7.6,8.,31.5));
#14207=CARTESIAN_POINT('Origin',(-4.4,8.,30.4));
#14208=CARTESIAN_POINT('',(-4.675,8.,30.5));
#14209=CARTESIAN_POINT('Origin',(-4.4,8.,30.5));
#14210=CARTESIAN_POINT('',(-4.675,8.,31.5));
#14211=CARTESIAN_POINT('',(-4.675,8.,30.4));
#14212=CARTESIAN_POINT('Origin',(-4.4,8.,31.5));
#14213=CARTESIAN_POINT('Origin',(-7.6,0.,30.4));
#14214=CARTESIAN_POINT('',(-7.875,-3.36777869765523E-17,30.5));
#14215=CARTESIAN_POINT('Origin',(-7.6,0.,30.5));
#14216=CARTESIAN_POINT('',(-7.875,3.36777869765523E-17,31.5));
#14217=CARTESIAN_POINT('',(-7.875,-3.36777869765523E-17,30.4));
#14218=CARTESIAN_POINT('Origin',(-7.6,0.,31.5));
#14219=CARTESIAN_POINT('Origin',(-4.4,0.,30.4));
#14220=CARTESIAN_POINT('',(-4.675,-3.36777869765523E-17,30.5));
#14221=CARTESIAN_POINT('Origin',(-4.4,0.,30.5));
#14222=CARTESIAN_POINT('',(-4.675,3.36777869765523E-17,31.5));
#14223=CARTESIAN_POINT('',(-4.675,-3.36777869765523E-17,30.4));
#14224=CARTESIAN_POINT('Origin',(-4.4,0.,31.5));
#14225=CARTESIAN_POINT('Origin',(9.5,10.,30.4));
#14226=CARTESIAN_POINT('',(9.225,10.,30.5));
#14227=CARTESIAN_POINT('Origin',(9.5,10.,30.5));
#14228=CARTESIAN_POINT('',(9.225,10.,31.5));
#14229=CARTESIAN_POINT('',(9.225,10.,30.4));
#14230=CARTESIAN_POINT('Origin',(9.5,10.,31.5));
#14231=CARTESIAN_POINT('Origin',(9.5,11.,30.4));
#14232=CARTESIAN_POINT('',(9.225,11.,30.5));
#14233=CARTESIAN_POINT('Origin',(9.5,11.,30.5));
#14234=CARTESIAN_POINT('',(9.225,11.,31.5));
#14235=CARTESIAN_POINT('',(9.225,11.,30.4));
#14236=CARTESIAN_POINT('Origin',(9.5,11.,31.5));
#14237=CARTESIAN_POINT('Origin',(-9.5,10.,30.4));
#14238=CARTESIAN_POINT('',(-9.775,10.,30.5));
#14239=CARTESIAN_POINT('Origin',(-9.5,10.,30.5));
#14240=CARTESIAN_POINT('',(-9.775,10.,31.5));
#14241=CARTESIAN_POINT('',(-9.775,10.,30.4));
#14242=CARTESIAN_POINT('Origin',(-9.5,10.,31.5));
#14243=CARTESIAN_POINT('Origin',(-9.5,11.,30.4));
#14244=CARTESIAN_POINT('',(-9.775,11.,30.5));
#14245=CARTESIAN_POINT('Origin',(-9.5,11.,30.5));
#14246=CARTESIAN_POINT('',(-9.775,11.,31.5));
#14247=CARTESIAN_POINT('',(-9.775,11.,30.4));
#14248=CARTESIAN_POINT('Origin',(-9.5,11.,31.5));
#14249=CARTESIAN_POINT('Origin',(6.,-4.,30.4));
#14250=CARTESIAN_POINT('',(5.39,-4.,30.5));
#14251=CARTESIAN_POINT('Origin',(6.,-4.,30.5));
#14252=CARTESIAN_POINT('',(5.39,-4.,31.5));
#14253=CARTESIAN_POINT('',(5.39,-4.,30.4));
#14254=CARTESIAN_POINT('Origin',(6.,-4.,31.5));
#14255=CARTESIAN_POINT('Origin',(-6.,4.,30.4));
#14256=CARTESIAN_POINT('',(-6.61,4.,30.5));
#14257=CARTESIAN_POINT('Origin',(-6.,4.,30.5));
#14258=CARTESIAN_POINT('',(-6.61,4.,31.5));
#14259=CARTESIAN_POINT('',(-6.61,4.,30.4));
#14260=CARTESIAN_POINT('Origin',(-6.,4.,31.5));
#14261=CARTESIAN_POINT('Origin',(-6.,-4.,30.4));
#14262=CARTESIAN_POINT('',(-6.61,-4.,30.5));
#14263=CARTESIAN_POINT('Origin',(-6.,-4.,30.5));
#14264=CARTESIAN_POINT('',(-6.61,-4.,31.5));
#14265=CARTESIAN_POINT('',(-6.61,-4.,30.4));
#14266=CARTESIAN_POINT('Origin',(-6.,-4.,31.5));
#14267=CARTESIAN_POINT('Origin',(6.,4.,30.4));
#14268=CARTESIAN_POINT('',(5.39,4.,30.5));
#14269=CARTESIAN_POINT('Origin',(6.,4.,30.5));
#14270=CARTESIAN_POINT('',(5.39,4.,31.5));
#14271=CARTESIAN_POINT('',(5.39,4.,30.4));
#14272=CARTESIAN_POINT('Origin',(6.,4.,31.5));
#14273=CARTESIAN_POINT('Origin',(10.5,11.5,30.5));
#14274=CARTESIAN_POINT('',(10.5,11.5,30.5));
#14275=CARTESIAN_POINT('',(-10.5,11.5,30.5));
#14276=CARTESIAN_POINT('',(10.5,11.5,30.5));
#14277=CARTESIAN_POINT('',(-10.5,11.5,31.5));
#14278=CARTESIAN_POINT('',(-10.5,11.5,30.5));
#14279=CARTESIAN_POINT('',(10.5,11.5,31.5));
#14280=CARTESIAN_POINT('',(10.5,11.5,31.5));
#14281=CARTESIAN_POINT('',(10.5,11.5,30.5));
#14282=CARTESIAN_POINT('Origin',(10.5,-8.,30.5));
#14283=CARTESIAN_POINT('',(10.5,-8.,30.5));
#14284=CARTESIAN_POINT('',(10.5,-8.,30.5));
#14285=CARTESIAN_POINT('',(10.5,-8.,31.5));
#14286=CARTESIAN_POINT('',(10.5,-8.,31.5));
#14287=CARTESIAN_POINT('',(10.5,-8.,30.5));
#14288=CARTESIAN_POINT('Origin',(-10.5,-8.,30.5));
#14289=CARTESIAN_POINT('',(-10.5,-8.,30.5));
#14290=CARTESIAN_POINT('',(-10.5,-8.,30.5));
#14291=CARTESIAN_POINT('',(-10.5,-8.,31.5));
#14292=CARTESIAN_POINT('',(-10.5,-8.,31.5));
#14293=CARTESIAN_POINT('',(-10.5,-8.,30.5));
#14294=CARTESIAN_POINT('Origin',(-10.5,11.5,30.5));
#14295=CARTESIAN_POINT('',(-10.5,11.5,30.5));
#14296=CARTESIAN_POINT('',(-10.5,11.5,31.5));
#14297=CARTESIAN_POINT('Origin',(0.,1.75,31.5));
#14298=CARTESIAN_POINT('Origin',(0.,1.75,30.5));
#22298=UNCERTAINTY_MEASURE_WITH_UNIT(LENGTH_MEASURE(0.001),#22395,
'DISTANCE_ACCURACY_VALUE',
'Maximum model space distance between geometric entities at asserted c
onnectivities');
#22343=UNCERTAINTY_MEASURE_WITH_UNIT(LENGTH_MEASURE(0.001),#22395,
'DISTANCE_ACCURACY_VALUE',
'Maximum model space distance between geometric entities at asserted c
onnectivities');
#22349=(
GEOMETRIC_REPRESENTATION_CONTEXT(3)
GLOBAL_UNCERTAINTY_ASSIGNED_CONTEXT((#22298))
GLOBAL_UNIT_ASSIGNED_CONTEXT((#22395,#22397,#22398))
REPRESENTATION_CONTEXT('','3D')
);
#22394=(
GEOMETRIC_REPRESENTATION_CONTEXT(3)
GLOBAL_UNCERTAINTY_ASSIGNED_CONTEXT((#22343))
GLOBAL_UNIT_ASSIGNED_CONTEXT((#22395,#22397,#22398))
REPRESENTATION_CONTEXT('','3D')
);
#22395=(
LENGTH_UNIT()
NAMED_UNIT(*)
SI_UNIT(.CENTI.,.METRE.)
);
#22397=(
NAMED_UNIT(*)
PLANE_ANGLE_UNIT()
SI_UNIT($,.RADIAN.)
);
#22398=(
NAMED_UNIT(*)
SI_UNIT($,.STERADIAN.)
SOLID_ANGLE_UNIT()
);
#22404=SHAPE_DEFINITION_REPRESENTATION(#22454,#22643);
#22454=PRODUCT_DEFINITION_SHAPE('',$,#22694);
#22643=SHAPE_REPRESENTATION('',(#9849),#22349);
#22688=PRODUCT_DEFINITION_CONTEXT('part definition',#22840,'design');
#22694=PRODUCT_DEFINITION('Guide header','Guide header',#22744,#22688);
#22744=PRODUCT_DEFINITION_FORMATION('',$,#22847);
#22840=APPLICATION_CONTEXT(
'Core Data for Automotive Mechanical Design Process');
#22841=PRODUCT_CONTEXT('part definition',#22840,'mechanical');
#22847=PRODUCT('Guide header','Guide header','Guide header',(#22841));
#22941=COLOUR_RGB('Light Blue',0.38,0.62,0.78);
#22942=FILL_AREA_STYLE_COLOUR('',#22941);
#22943=FILL_AREA_STYLE('',(#22942));
#22944=SURFACE_STYLE_FILL_AREA(#22943);
#22945=SURFACE_SIDE_STYLE('',(#22944));
#22946=SURFACE_STYLE_USAGE(.BOTH.,#22945);
#22947=PRESENTATION_STYLE_ASSIGNMENT((#22946));
ENDSEC;
END-ISO-10303-21;
